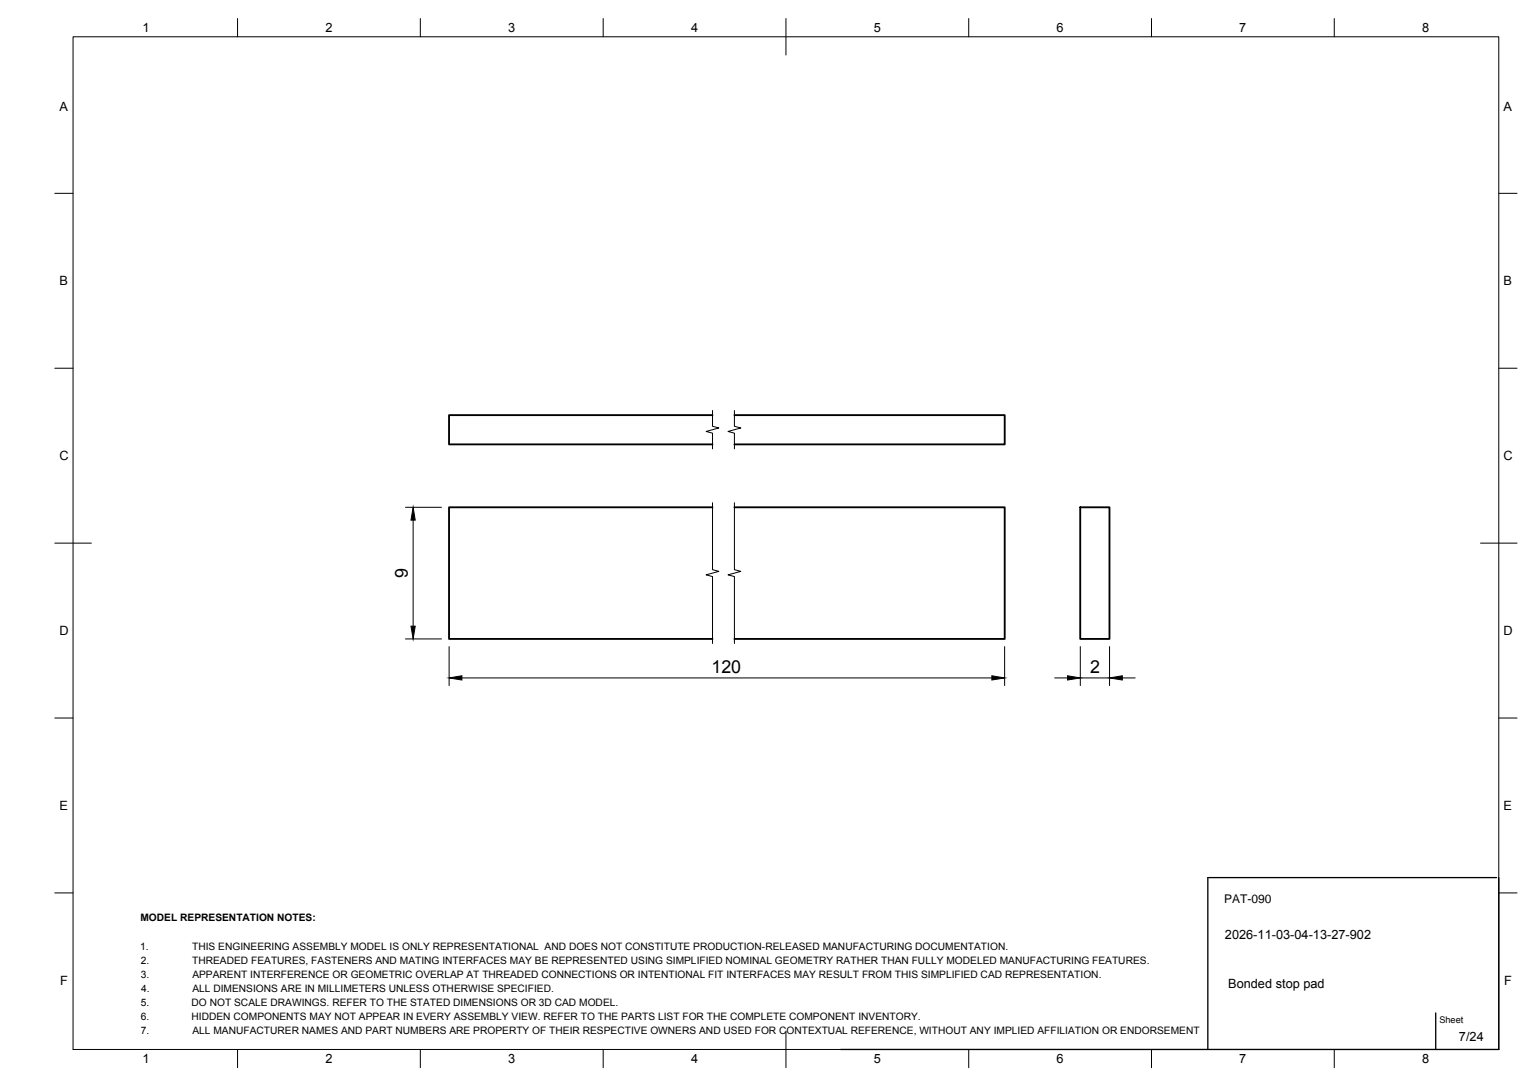
ISO-10303-21;
HEADER;
/* Generated by software containing ST-Developer
 * from STEP Tools, Inc. (www.steptools.com) 
 */

FILE_DESCRIPTION(
/* description */ ('Round-Shaft Linear Stage with Ball Bushings'),
/* implementation_level */ '2;1');

FILE_NAME(
/* name */ 'Bonded stop pad.step',
/* time_stamp */ '2026-10-27T10:47:55-07:00',
/* author */ (''),
/* organization */ (''),
/* preprocessor_version */ 'ST-DEVELOPER v20.2',
/* originating_system */ 'Autodesk Translation Framework v15.17.0.0',
/* authorisation */ '');

FILE_SCHEMA (('AUTOMOTIVE_DESIGN { 1 0 10303 214 3 1 1 }'));
ENDSEC;

DATA;
#10=MECHANICAL_DESIGN_GEOMETRIC_PRESENTATION_REPRESENTATION('',(#304),#7835);
#262=SHAPE_REPRESENTATION_RELATIONSHIP('SRR','None',#7950,#283);
#283=ADVANCED_BREP_SHAPE_REPRESENTATION('',(#325),#7814);
#304=STYLED_ITEM('',(#8158),#325);
#325=MANIFOLD_SOLID_BREP('Body1',#4394);
#473=PLANE('',#4716);
#474=PLANE('',#4717);
#475=PLANE('',#4718);
#476=PLANE('',#4719);
#477=PLANE('',#4720);
#478=PLANE('',#4721);
#646=FACE_OUTER_BOUND('',#933,.T.);
#647=FACE_OUTER_BOUND('',#934,.T.);
#648=FACE_OUTER_BOUND('',#935,.T.);
#649=FACE_OUTER_BOUND('',#936,.T.);
#650=FACE_OUTER_BOUND('',#937,.T.);
#651=FACE_OUTER_BOUND('',#938,.T.);
#933=EDGE_LOOP('',(#3138,#3139,#3140,#3141));
#934=EDGE_LOOP('',(#3142,#3143,#3144,#3145));
#935=EDGE_LOOP('',(#3146,#3147,#3148,#3149));
#936=EDGE_LOOP('',(#3150,#3151,#3152,#3153));
#937=EDGE_LOOP('',(#3154,#3155,#3156,#3157));
#938=EDGE_LOOP('',(#3158,#3159,#3160,#3161));
#1289=LINE('',#6728,#1629);
#1290=LINE('',#6730,#1630);
#1291=LINE('',#6732,#1631);
#1292=LINE('',#6733,#1632);
#1293=LINE('',#6736,#1633);
#1294=LINE('',#6738,#1634);
#1295=LINE('',#6739,#1635);
#1296=LINE('',#6742,#1636);
#1297=LINE('',#6744,#1637);
#1298=LINE('',#6745,#1638);
#1299=LINE('',#6747,#1639);
#1300=LINE('',#6748,#1640);
#1629=VECTOR('',#5352,1.);
#1630=VECTOR('',#5353,1.);
#1631=VECTOR('',#5354,1.);
#1632=VECTOR('',#5355,1.);
#1633=VECTOR('',#5358,1.);
#1634=VECTOR('',#5359,1.);
#1635=VECTOR('',#5360,1.);
#1636=VECTOR('',#5363,1.);
#1637=VECTOR('',#5364,1.);
#1638=VECTOR('',#5365,1.);
#1639=VECTOR('',#5368,1.);
#1640=VECTOR('',#5369,1.);
#2166=VERTEX_POINT('',#6726);
#2167=VERTEX_POINT('',#6727);
#2168=VERTEX_POINT('',#6729);
#2169=VERTEX_POINT('',#6731);
#2170=VERTEX_POINT('',#6735);
#2171=VERTEX_POINT('',#6737);
#2172=VERTEX_POINT('',#6741);
#2173=VERTEX_POINT('',#6743);
#2537=EDGE_CURVE('',#2166,#2167,#1289,.T.);
#2538=EDGE_CURVE('',#2167,#2168,#1290,.T.);
#2539=EDGE_CURVE('',#2169,#2168,#1291,.T.);
#2540=EDGE_CURVE('',#2166,#2169,#1292,.T.);
#2541=EDGE_CURVE('',#2170,#2166,#1293,.T.);
#2542=EDGE_CURVE('',#2171,#2169,#1294,.T.);
#2543=EDGE_CURVE('',#2170,#2171,#1295,.T.);
#2544=EDGE_CURVE('',#2172,#2170,#1296,.T.);
#2545=EDGE_CURVE('',#2173,#2171,#1297,.T.);
#2546=EDGE_CURVE('',#2172,#2173,#1298,.T.);
#2547=EDGE_CURVE('',#2167,#2172,#1299,.T.);
#2548=EDGE_CURVE('',#2168,#2173,#1300,.T.);
#3138=ORIENTED_EDGE('',*,*,#2537,.T.);
#3139=ORIENTED_EDGE('',*,*,#2538,.T.);
#3140=ORIENTED_EDGE('',*,*,#2539,.F.);
#3141=ORIENTED_EDGE('',*,*,#2540,.F.);
#3142=ORIENTED_EDGE('',*,*,#2541,.T.);
#3143=ORIENTED_EDGE('',*,*,#2540,.T.);
#3144=ORIENTED_EDGE('',*,*,#2542,.F.);
#3145=ORIENTED_EDGE('',*,*,#2543,.F.);
#3146=ORIENTED_EDGE('',*,*,#2544,.T.);
#3147=ORIENTED_EDGE('',*,*,#2543,.T.);
#3148=ORIENTED_EDGE('',*,*,#2545,.F.);
#3149=ORIENTED_EDGE('',*,*,#2546,.F.);
#3150=ORIENTED_EDGE('',*,*,#2547,.T.);
#3151=ORIENTED_EDGE('',*,*,#2546,.T.);
#3152=ORIENTED_EDGE('',*,*,#2548,.F.);
#3153=ORIENTED_EDGE('',*,*,#2538,.F.);
#3154=ORIENTED_EDGE('',*,*,#2548,.T.);
#3155=ORIENTED_EDGE('',*,*,#2545,.T.);
#3156=ORIENTED_EDGE('',*,*,#2542,.T.);
#3157=ORIENTED_EDGE('',*,*,#2539,.T.);
#3158=ORIENTED_EDGE('',*,*,#2547,.F.);
#3159=ORIENTED_EDGE('',*,*,#2537,.F.);
#3160=ORIENTED_EDGE('',*,*,#2541,.F.);
#3161=ORIENTED_EDGE('',*,*,#2544,.F.);
#4165=ADVANCED_FACE('',(#646),#473,.T.);
#4166=ADVANCED_FACE('',(#647),#474,.T.);
#4167=ADVANCED_FACE('',(#648),#475,.T.);
#4168=ADVANCED_FACE('',(#649),#476,.T.);
#4169=ADVANCED_FACE('',(#650),#477,.T.);
#4170=ADVANCED_FACE('',(#651),#478,.F.);
#4394=CLOSED_SHELL('',(#4165,#4166,#4167,#4168,#4169,#4170));
#4715=AXIS2_PLACEMENT_3D('',#6724,#5348,#5349);
#4716=AXIS2_PLACEMENT_3D('',#6725,#5350,#5351);
#4717=AXIS2_PLACEMENT_3D('',#6734,#5356,#5357);
#4718=AXIS2_PLACEMENT_3D('',#6740,#5361,#5362);
#4719=AXIS2_PLACEMENT_3D('',#6746,#5366,#5367);
#4720=AXIS2_PLACEMENT_3D('',#6749,#5370,#5371);
#4721=AXIS2_PLACEMENT_3D('',#6750,#5372,#5373);
#5348=DIRECTION('axis',(0.,0.,1.));
#5349=DIRECTION('refdir',(1.,0.,0.));
#5350=DIRECTION('center_axis',(0.,1.,0.));
#5351=DIRECTION('ref_axis',(-1.,0.,0.));
#5352=DIRECTION('',(-1.,0.,0.));
#5353=DIRECTION('',(0.,0.,1.));
#5354=DIRECTION('',(-1.,0.,0.));
#5355=DIRECTION('',(0.,0.,1.));
#5356=DIRECTION('center_axis',(1.,0.,0.));
#5357=DIRECTION('ref_axis',(0.,1.,0.));
#5358=DIRECTION('',(0.,1.,0.));
#5359=DIRECTION('',(0.,1.,0.));
#5360=DIRECTION('',(0.,0.,1.));
#5361=DIRECTION('center_axis',(0.,-1.,0.));
#5362=DIRECTION('ref_axis',(1.,0.,0.));
#5363=DIRECTION('',(1.,0.,0.));
#5364=DIRECTION('',(1.,0.,0.));
#5365=DIRECTION('',(0.,0.,1.));
#5366=DIRECTION('center_axis',(-1.,0.,0.));
#5367=DIRECTION('ref_axis',(0.,-1.,0.));
#5368=DIRECTION('',(0.,-1.,0.));
#5369=DIRECTION('',(0.,-1.,0.));
#5370=DIRECTION('center_axis',(0.,0.,1.));
#5371=DIRECTION('ref_axis',(1.,0.,0.));
#5372=DIRECTION('center_axis',(0.,0.,1.));
#5373=DIRECTION('ref_axis',(1.,0.,0.));
#6724=CARTESIAN_POINT('',(0.,0.,0.));
#6725=CARTESIAN_POINT('Origin',(4.2,6.,1.6));
#6726=CARTESIAN_POINT('',(4.2,6.,1.6));
#6727=CARTESIAN_POINT('',(4.,6.,1.6));
#6728=CARTESIAN_POINT('',(4.2,6.,1.6));
#6729=CARTESIAN_POINT('',(4.,6.,2.5));
#6730=CARTESIAN_POINT('',(4.,6.,1.6));
#6731=CARTESIAN_POINT('',(4.2,6.,2.5));
#6732=CARTESIAN_POINT('',(4.2,6.,2.5));
#6733=CARTESIAN_POINT('',(4.2,6.,1.6));
#6734=CARTESIAN_POINT('Origin',(4.2,-6.,1.6));
#6735=CARTESIAN_POINT('',(4.2,-6.,1.6));
#6736=CARTESIAN_POINT('',(4.2,-6.,1.6));
#6737=CARTESIAN_POINT('',(4.2,-6.,2.5));
#6738=CARTESIAN_POINT('',(4.2,-6.,2.5));
#6739=CARTESIAN_POINT('',(4.2,-6.,1.6));
#6740=CARTESIAN_POINT('Origin',(4.,-6.,1.6));
#6741=CARTESIAN_POINT('',(4.,-6.,1.6));
#6742=CARTESIAN_POINT('',(4.,-6.,1.6));
#6743=CARTESIAN_POINT('',(4.,-6.,2.5));
#6744=CARTESIAN_POINT('',(4.,-6.,2.5));
#6745=CARTESIAN_POINT('',(4.,-6.,1.6));
#6746=CARTESIAN_POINT('Origin',(4.,6.,1.6));
#6747=CARTESIAN_POINT('',(4.,6.,1.6));
#6748=CARTESIAN_POINT('',(4.,6.,2.5));
#6749=CARTESIAN_POINT('Origin',(4.1,0.,2.5));
#6750=CARTESIAN_POINT('Origin',(4.1,0.,1.6));
#7788=UNCERTAINTY_MEASURE_WITH_UNIT(LENGTH_MEASURE(0.001),#7836,
'DISTANCE_ACCURACY_VALUE',
'Maximum model space distance between geometric entities at asserted c
onnectivities');
#7809=UNCERTAINTY_MEASURE_WITH_UNIT(LENGTH_MEASURE(0.001),#7836,
'DISTANCE_ACCURACY_VALUE',
'Maximum model space distance between geometric entities at asserted c
onnectivities');
#7814=(
GEOMETRIC_REPRESENTATION_CONTEXT(3)
GLOBAL_UNCERTAINTY_ASSIGNED_CONTEXT((#7788))
GLOBAL_UNIT_ASSIGNED_CONTEXT((#7836,#7838,#7839))
REPRESENTATION_CONTEXT('','3D')
);
#7835=(
GEOMETRIC_REPRESENTATION_CONTEXT(3)
GLOBAL_UNCERTAINTY_ASSIGNED_CONTEXT((#7809))
GLOBAL_UNIT_ASSIGNED_CONTEXT((#7836,#7838,#7839))
REPRESENTATION_CONTEXT('','3D')
);
#7836=(
LENGTH_UNIT()
NAMED_UNIT(*)
SI_UNIT(.CENTI.,.METRE.)
);
#7838=(
NAMED_UNIT(*)
PLANE_ANGLE_UNIT()
SI_UNIT($,.RADIAN.)
);
#7839=(
NAMED_UNIT(*)
SI_UNIT($,.STERADIAN.)
SOLID_ANGLE_UNIT()
);
#7844=SHAPE_DEFINITION_REPRESENTATION(#7869,#7950);
#7869=PRODUCT_DEFINITION_SHAPE('',$,#7976);
#7950=SHAPE_REPRESENTATION('',(#4715),#7814);
#7971=PRODUCT_DEFINITION_CONTEXT('part definition',#8048,'design');
#7976=PRODUCT_DEFINITION('Bonded stop pad','Bonded stop pad',#8001,#7971);
#8001=PRODUCT_DEFINITION_FORMATION('',$,#8054);
#8048=APPLICATION_CONTEXT(
'Core Data for Automotive Mechanical Design Process');
#8049=PRODUCT_CONTEXT('part definition',#8048,'mechanical');
#8054=PRODUCT('Bonded stop pad','Bonded stop pad','Bonded stop pad',(#8049));
#8152=COLOUR_RGB('Off White',0.89,0.88,0.83);
#8153=FILL_AREA_STYLE_COLOUR('',#8152);
#8154=FILL_AREA_STYLE('',(#8153));
#8155=SURFACE_STYLE_FILL_AREA(#8154);
#8156=SURFACE_SIDE_STYLE('',(#8155));
#8157=SURFACE_STYLE_USAGE(.BOTH.,#8156);
#8158=PRESENTATION_STYLE_ASSIGNMENT((#8157));
ENDSEC;
END-ISO-10303-21;
